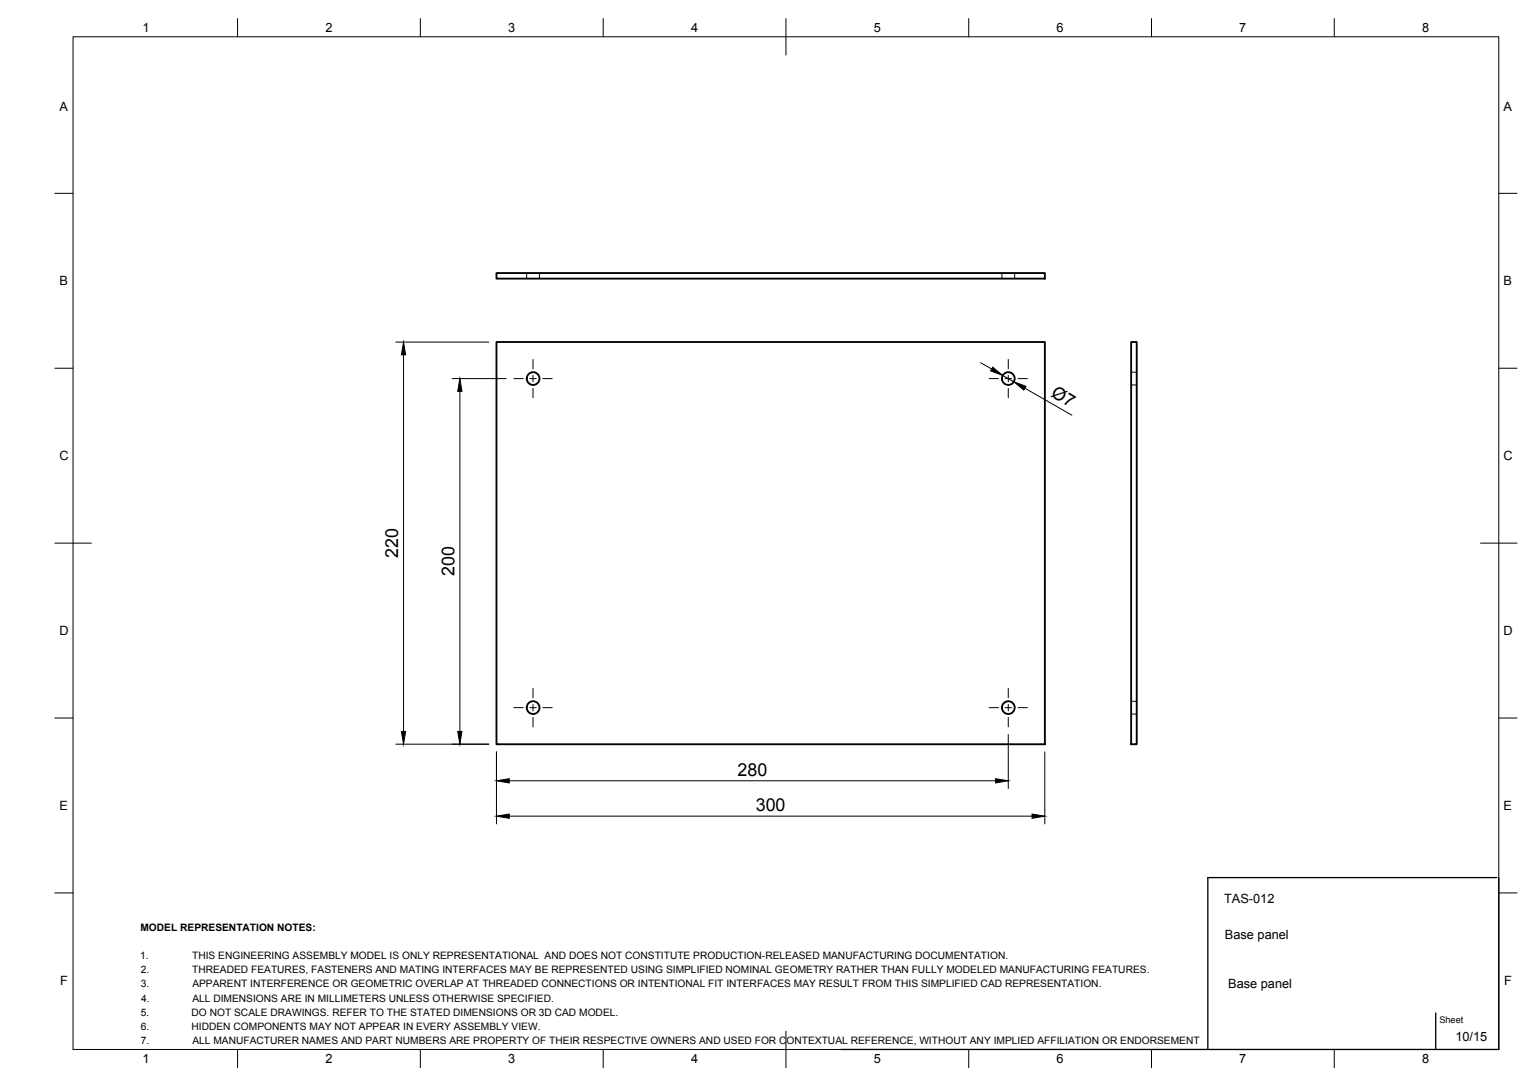
ISO-10303-21;
HEADER;
/* Generated by software containing ST-Developer
 * from STEP Tools, Inc. (www.steptools.com) 
 */

FILE_DESCRIPTION(
/* description */ (
'Independent welded steel electronics enclosure with removable sealed 
lid, internal mounting tray and two threaded cable entries. 300 x 220 
mm body. No ingress or electrical safety rating assigned.'),
/* implementation_level */ '2;1');

FILE_NAME(
/* name */ 'Base panel.step',
/* time_stamp */ '2026-11-14T09:13:27-08:00',
/* author */ (''),
/* organization */ (''),
/* preprocessor_version */ 'ST-DEVELOPER v20.2',
/* originating_system */ 'Autodesk Translation Framework v15.17.0.0',
/* authorisation */ '');

FILE_SCHEMA (('AUTOMOTIVE_DESIGN { 1 0 10303 214 3 1 1 }'));
ENDSEC;

DATA;
#10=MECHANICAL_DESIGN_GEOMETRIC_PRESENTATION_REPRESENTATION('',(#966),#94412);
#936=SHAPE_REPRESENTATION_RELATIONSHIP('SRR','None',#94488,#951);
#951=ADVANCED_BREP_SHAPE_REPRESENTATION('',(#981),#94397);
#966=STYLED_ITEM('',(#94576),#981);
#981=MANIFOLD_SOLID_BREP('Body1',#8251);
#996=FACE_BOUND('',#1523,.T.);
#997=FACE_BOUND('',#1524,.T.);
#998=FACE_BOUND('',#1525,.T.);
#999=FACE_BOUND('',#1526,.T.);
#1000=FACE_BOUND('',#1528,.T.);
#1001=FACE_BOUND('',#1529,.T.);
#1002=FACE_BOUND('',#1530,.T.);
#1003=FACE_BOUND('',#1531,.T.);
#1058=PLANE('',#8447);
#1059=PLANE('',#8448);
#1060=PLANE('',#8449);
#1061=PLANE('',#8450);
#1062=PLANE('',#8451);
#1063=PLANE('',#8452);
#1158=FACE_OUTER_BOUND('',#1514,.T.);
#1159=FACE_OUTER_BOUND('',#1515,.T.);
#1160=FACE_OUTER_BOUND('',#1516,.T.);
#1161=FACE_OUTER_BOUND('',#1517,.T.);
#1162=FACE_OUTER_BOUND('',#1518,.T.);
#1163=FACE_OUTER_BOUND('',#1519,.T.);
#1164=FACE_OUTER_BOUND('',#1520,.T.);
#1165=FACE_OUTER_BOUND('',#1521,.T.);
#1166=FACE_OUTER_BOUND('',#1522,.T.);
#1167=FACE_OUTER_BOUND('',#1527,.T.);
#1514=EDGE_LOOP('',(#5094,#5095,#5096,#5097));
#1515=EDGE_LOOP('',(#5098,#5099,#5100,#5101));
#1516=EDGE_LOOP('',(#5102,#5103,#5104,#5105));
#1517=EDGE_LOOP('',(#5106,#5107,#5108,#5109));
#1518=EDGE_LOOP('',(#5110,#5111,#5112,#5113));
#1519=EDGE_LOOP('',(#5114,#5115,#5116,#5117));
#1520=EDGE_LOOP('',(#5118,#5119,#5120,#5121));
#1521=EDGE_LOOP('',(#5122,#5123,#5124,#5125));
#1522=EDGE_LOOP('',(#5126,#5127,#5128,#5129));
#1523=EDGE_LOOP('',(#5130));
#1524=EDGE_LOOP('',(#5131));
#1525=EDGE_LOOP('',(#5132));
#1526=EDGE_LOOP('',(#5133));
#1527=EDGE_LOOP('',(#5134,#5135,#5136,#5137));
#1528=EDGE_LOOP('',(#5138));
#1529=EDGE_LOOP('',(#5139));
#1530=EDGE_LOOP('',(#5140));
#1531=EDGE_LOOP('',(#5141));
#1932=LINE('',#10367,#2330);
#1933=LINE('',#10373,#2331);
#1934=LINE('',#10379,#2332);
#1935=LINE('',#10385,#2333);
#1936=LINE('',#10390,#2334);
#1937=LINE('',#10392,#2335);
#1938=LINE('',#10394,#2336);
#1939=LINE('',#10395,#2337);
#1940=LINE('',#10398,#2338);
#1941=LINE('',#10400,#2339);
#1942=LINE('',#10401,#2340);
#1943=LINE('',#10404,#2341);
#1944=LINE('',#10406,#2342);
#1945=LINE('',#10407,#2343);
#1946=LINE('',#10409,#2344);
#1947=LINE('',#10410,#2345);
#2330=VECTOR('',#8952,3.5);
#2331=VECTOR('',#8959,3.5);
#2332=VECTOR('',#8966,3.5);
#2333=VECTOR('',#8973,3.5);
#2334=VECTOR('',#8978,10.);
#2335=VECTOR('',#8979,10.);
#2336=VECTOR('',#8980,10.);
#2337=VECTOR('',#8981,10.);
#2338=VECTOR('',#8984,10.);
#2339=VECTOR('',#8985,10.);
#2340=VECTOR('',#8986,10.);
#2341=VECTOR('',#8989,10.);
#2342=VECTOR('',#8990,10.);
#2343=VECTOR('',#8991,10.);
#2344=VECTOR('',#8994,10.);
#2345=VECTOR('',#8995,10.);
#2728=CIRCLE('',#8436,3.5);
#2729=CIRCLE('',#8437,3.5);
#2730=CIRCLE('',#8439,3.5);
#2731=CIRCLE('',#8440,3.5);
#2732=CIRCLE('',#8442,3.5);
#2733=CIRCLE('',#8443,3.5);
#2734=CIRCLE('',#8445,3.5);
#2735=CIRCLE('',#8446,3.5);
#2846=VERTEX_POINT('',#10364);
#2847=VERTEX_POINT('',#10366);
#2848=VERTEX_POINT('',#10370);
#2849=VERTEX_POINT('',#10372);
#2850=VERTEX_POINT('',#10376);
#2851=VERTEX_POINT('',#10378);
#2852=VERTEX_POINT('',#10382);
#2853=VERTEX_POINT('',#10384);
#2854=VERTEX_POINT('',#10388);
#2855=VERTEX_POINT('',#10389);
#2856=VERTEX_POINT('',#10391);
#2857=VERTEX_POINT('',#10393);
#2858=VERTEX_POINT('',#10397);
#2859=VERTEX_POINT('',#10399);
#2860=VERTEX_POINT('',#10403);
#2861=VERTEX_POINT('',#10405);
#3812=EDGE_CURVE('',#2846,#2846,#2728,.T.);
#3813=EDGE_CURVE('',#2846,#2847,#1932,.T.);
#3814=EDGE_CURVE('',#2847,#2847,#2729,.T.);
#3815=EDGE_CURVE('',#2848,#2848,#2730,.T.);
#3816=EDGE_CURVE('',#2848,#2849,#1933,.T.);
#3817=EDGE_CURVE('',#2849,#2849,#2731,.T.);
#3818=EDGE_CURVE('',#2850,#2850,#2732,.T.);
#3819=EDGE_CURVE('',#2850,#2851,#1934,.T.);
#3820=EDGE_CURVE('',#2851,#2851,#2733,.T.);
#3821=EDGE_CURVE('',#2852,#2852,#2734,.T.);
#3822=EDGE_CURVE('',#2852,#2853,#1935,.T.);
#3823=EDGE_CURVE('',#2853,#2853,#2735,.T.);
#3824=EDGE_CURVE('',#2854,#2855,#1936,.T.);
#3825=EDGE_CURVE('',#2855,#2856,#1937,.T.);
#3826=EDGE_CURVE('',#2857,#2856,#1938,.T.);
#3827=EDGE_CURVE('',#2854,#2857,#1939,.T.);
#3828=EDGE_CURVE('',#2858,#2854,#1940,.T.);
#3829=EDGE_CURVE('',#2859,#2857,#1941,.T.);
#3830=EDGE_CURVE('',#2858,#2859,#1942,.T.);
#3831=EDGE_CURVE('',#2860,#2858,#1943,.T.);
#3832=EDGE_CURVE('',#2861,#2859,#1944,.T.);
#3833=EDGE_CURVE('',#2860,#2861,#1945,.T.);
#3834=EDGE_CURVE('',#2855,#2860,#1946,.T.);
#3835=EDGE_CURVE('',#2856,#2861,#1947,.T.);
#5094=ORIENTED_EDGE('',*,*,#3812,.F.);
#5095=ORIENTED_EDGE('',*,*,#3813,.T.);
#5096=ORIENTED_EDGE('',*,*,#3814,.F.);
#5097=ORIENTED_EDGE('',*,*,#3813,.F.);
#5098=ORIENTED_EDGE('',*,*,#3815,.F.);
#5099=ORIENTED_EDGE('',*,*,#3816,.T.);
#5100=ORIENTED_EDGE('',*,*,#3817,.F.);
#5101=ORIENTED_EDGE('',*,*,#3816,.F.);
#5102=ORIENTED_EDGE('',*,*,#3818,.F.);
#5103=ORIENTED_EDGE('',*,*,#3819,.T.);
#5104=ORIENTED_EDGE('',*,*,#3820,.F.);
#5105=ORIENTED_EDGE('',*,*,#3819,.F.);
#5106=ORIENTED_EDGE('',*,*,#3821,.F.);
#5107=ORIENTED_EDGE('',*,*,#3822,.T.);
#5108=ORIENTED_EDGE('',*,*,#3823,.F.);
#5109=ORIENTED_EDGE('',*,*,#3822,.F.);
#5110=ORIENTED_EDGE('',*,*,#3824,.T.);
#5111=ORIENTED_EDGE('',*,*,#3825,.T.);
#5112=ORIENTED_EDGE('',*,*,#3826,.F.);
#5113=ORIENTED_EDGE('',*,*,#3827,.F.);
#5114=ORIENTED_EDGE('',*,*,#3828,.T.);
#5115=ORIENTED_EDGE('',*,*,#3827,.T.);
#5116=ORIENTED_EDGE('',*,*,#3829,.F.);
#5117=ORIENTED_EDGE('',*,*,#3830,.F.);
#5118=ORIENTED_EDGE('',*,*,#3831,.T.);
#5119=ORIENTED_EDGE('',*,*,#3830,.T.);
#5120=ORIENTED_EDGE('',*,*,#3832,.F.);
#5121=ORIENTED_EDGE('',*,*,#3833,.F.);
#5122=ORIENTED_EDGE('',*,*,#3834,.T.);
#5123=ORIENTED_EDGE('',*,*,#3833,.T.);
#5124=ORIENTED_EDGE('',*,*,#3835,.F.);
#5125=ORIENTED_EDGE('',*,*,#3825,.F.);
#5126=ORIENTED_EDGE('',*,*,#3835,.T.);
#5127=ORIENTED_EDGE('',*,*,#3832,.T.);
#5128=ORIENTED_EDGE('',*,*,#3829,.T.);
#5129=ORIENTED_EDGE('',*,*,#3826,.T.);
#5130=ORIENTED_EDGE('',*,*,#3812,.T.);
#5131=ORIENTED_EDGE('',*,*,#3815,.T.);
#5132=ORIENTED_EDGE('',*,*,#3818,.T.);
#5133=ORIENTED_EDGE('',*,*,#3821,.T.);
#5134=ORIENTED_EDGE('',*,*,#3834,.F.);
#5135=ORIENTED_EDGE('',*,*,#3824,.F.);
#5136=ORIENTED_EDGE('',*,*,#3828,.F.);
#5137=ORIENTED_EDGE('',*,*,#3831,.F.);
#5138=ORIENTED_EDGE('',*,*,#3814,.T.);
#5139=ORIENTED_EDGE('',*,*,#3817,.T.);
#5140=ORIENTED_EDGE('',*,*,#3820,.T.);
#5141=ORIENTED_EDGE('',*,*,#3823,.T.);
#7658=CYLINDRICAL_SURFACE('',#8435,3.5);
#7659=CYLINDRICAL_SURFACE('',#8438,3.5);
#7660=CYLINDRICAL_SURFACE('',#8441,3.5);
#7661=CYLINDRICAL_SURFACE('',#8444,3.5);
#7895=ADVANCED_FACE('',(#1158),#7658,.F.);
#7896=ADVANCED_FACE('',(#1159),#7659,.F.);
#7897=ADVANCED_FACE('',(#1160),#7660,.F.);
#7898=ADVANCED_FACE('',(#1161),#7661,.F.);
#7899=ADVANCED_FACE('',(#1162),#1058,.T.);
#7900=ADVANCED_FACE('',(#1163),#1059,.T.);
#7901=ADVANCED_FACE('',(#1164),#1060,.T.);
#7902=ADVANCED_FACE('',(#1165),#1061,.T.);
#7903=ADVANCED_FACE('',(#1166,#996,#997,#998,#999),#1062,.T.);
#7904=ADVANCED_FACE('',(#1167,#1000,#1001,#1002,#1003),#1063,.F.);
#8251=CLOSED_SHELL('',(#7895,#7896,#7897,#7898,#7899,#7900,#7901,#7902,
#7903,#7904));
#8434=AXIS2_PLACEMENT_3D('',#10362,#8946,#8947);
#8435=AXIS2_PLACEMENT_3D('',#10363,#8948,#8949);
#8436=AXIS2_PLACEMENT_3D('',#10365,#8950,#8951);
#8437=AXIS2_PLACEMENT_3D('',#10368,#8953,#8954);
#8438=AXIS2_PLACEMENT_3D('',#10369,#8955,#8956);
#8439=AXIS2_PLACEMENT_3D('',#10371,#8957,#8958);
#8440=AXIS2_PLACEMENT_3D('',#10374,#8960,#8961);
#8441=AXIS2_PLACEMENT_3D('',#10375,#8962,#8963);
#8442=AXIS2_PLACEMENT_3D('',#10377,#8964,#8965);
#8443=AXIS2_PLACEMENT_3D('',#10380,#8967,#8968);
#8444=AXIS2_PLACEMENT_3D('',#10381,#8969,#8970);
#8445=AXIS2_PLACEMENT_3D('',#10383,#8971,#8972);
#8446=AXIS2_PLACEMENT_3D('',#10386,#8974,#8975);
#8447=AXIS2_PLACEMENT_3D('',#10387,#8976,#8977);
#8448=AXIS2_PLACEMENT_3D('',#10396,#8982,#8983);
#8449=AXIS2_PLACEMENT_3D('',#10402,#8987,#8988);
#8450=AXIS2_PLACEMENT_3D('',#10408,#8992,#8993);
#8451=AXIS2_PLACEMENT_3D('',#10411,#8996,#8997);
#8452=AXIS2_PLACEMENT_3D('',#10412,#8998,#8999);
#8946=DIRECTION('axis',(0.,0.,1.));
#8947=DIRECTION('refdir',(1.,0.,0.));
#8948=DIRECTION('center_axis',(0.,0.,-1.));
#8949=DIRECTION('ref_axis',(1.,0.,0.));
#8950=DIRECTION('center_axis',(0.,0.,-1.));
#8951=DIRECTION('ref_axis',(1.,0.,0.));
#8952=DIRECTION('',(0.,0.,-1.));
#8953=DIRECTION('center_axis',(0.,0.,1.));
#8954=DIRECTION('ref_axis',(1.,0.,0.));
#8955=DIRECTION('center_axis',(0.,0.,-1.));
#8956=DIRECTION('ref_axis',(1.,0.,0.));
#8957=DIRECTION('center_axis',(0.,0.,-1.));
#8958=DIRECTION('ref_axis',(1.,0.,0.));
#8959=DIRECTION('',(0.,0.,-1.));
#8960=DIRECTION('center_axis',(0.,0.,1.));
#8961=DIRECTION('ref_axis',(1.,0.,0.));
#8962=DIRECTION('center_axis',(0.,0.,-1.));
#8963=DIRECTION('ref_axis',(1.,0.,0.));
#8964=DIRECTION('center_axis',(0.,0.,-1.));
#8965=DIRECTION('ref_axis',(1.,0.,0.));
#8966=DIRECTION('',(0.,0.,-1.));
#8967=DIRECTION('center_axis',(0.,0.,1.));
#8968=DIRECTION('ref_axis',(1.,0.,0.));
#8969=DIRECTION('center_axis',(0.,0.,-1.));
#8970=DIRECTION('ref_axis',(1.,0.,0.));
#8971=DIRECTION('center_axis',(0.,0.,-1.));
#8972=DIRECTION('ref_axis',(1.,0.,0.));
#8973=DIRECTION('',(0.,0.,-1.));
#8974=DIRECTION('center_axis',(0.,0.,1.));
#8975=DIRECTION('ref_axis',(1.,0.,0.));
#8976=DIRECTION('center_axis',(0.,1.,0.));
#8977=DIRECTION('ref_axis',(-1.,0.,0.));
#8978=DIRECTION('',(-1.,0.,0.));
#8979=DIRECTION('',(0.,0.,1.));
#8980=DIRECTION('',(-1.,0.,0.));
#8981=DIRECTION('',(0.,0.,1.));
#8982=DIRECTION('center_axis',(1.,0.,0.));
#8983=DIRECTION('ref_axis',(0.,1.,0.));
#8984=DIRECTION('',(0.,1.,0.));
#8985=DIRECTION('',(0.,1.,0.));
#8986=DIRECTION('',(0.,0.,1.));
#8987=DIRECTION('center_axis',(0.,-1.,0.));
#8988=DIRECTION('ref_axis',(1.,0.,0.));
#8989=DIRECTION('',(1.,0.,0.));
#8990=DIRECTION('',(1.,0.,0.));
#8991=DIRECTION('',(0.,0.,1.));
#8992=DIRECTION('center_axis',(-1.,0.,0.));
#8993=DIRECTION('ref_axis',(0.,-1.,0.));
#8994=DIRECTION('',(0.,-1.,0.));
#8995=DIRECTION('',(0.,-1.,0.));
#8996=DIRECTION('center_axis',(0.,0.,1.));
#8997=DIRECTION('ref_axis',(1.,0.,0.));
#8998=DIRECTION('center_axis',(0.,0.,1.));
#8999=DIRECTION('ref_axis',(1.,0.,0.));
#10362=CARTESIAN_POINT('',(0.,0.,0.));
#10363=CARTESIAN_POINT('Origin',(130.,-90.,1.5));
#10364=CARTESIAN_POINT('',(126.5,-90.,3.));
#10365=CARTESIAN_POINT('Origin',(130.,-90.,3.));
#10366=CARTESIAN_POINT('',(126.5,-90.,0.));
#10367=CARTESIAN_POINT('',(126.5,-90.,1.5));
#10368=CARTESIAN_POINT('Origin',(130.,-90.,0.));
#10369=CARTESIAN_POINT('Origin',(-130.,-90.,1.5));
#10370=CARTESIAN_POINT('',(-133.5,-90.,3.));
#10371=CARTESIAN_POINT('Origin',(-130.,-90.,3.));
#10372=CARTESIAN_POINT('',(-133.5,-90.,0.));
#10373=CARTESIAN_POINT('',(-133.5,-90.,1.5));
#10374=CARTESIAN_POINT('Origin',(-130.,-90.,0.));
#10375=CARTESIAN_POINT('Origin',(-130.,90.,1.5));
#10376=CARTESIAN_POINT('',(-133.5,90.,3.));
#10377=CARTESIAN_POINT('Origin',(-130.,90.,3.));
#10378=CARTESIAN_POINT('',(-133.5,90.,0.));
#10379=CARTESIAN_POINT('',(-133.5,90.,1.5));
#10380=CARTESIAN_POINT('Origin',(-130.,90.,0.));
#10381=CARTESIAN_POINT('Origin',(130.,90.,1.5));
#10382=CARTESIAN_POINT('',(126.5,90.,3.));
#10383=CARTESIAN_POINT('Origin',(130.,90.,3.));
#10384=CARTESIAN_POINT('',(126.5,90.,0.));
#10385=CARTESIAN_POINT('',(126.5,90.,1.5));
#10386=CARTESIAN_POINT('Origin',(130.,90.,0.));
#10387=CARTESIAN_POINT('Origin',(150.,110.,0.));
#10388=CARTESIAN_POINT('',(150.,110.,0.));
#10389=CARTESIAN_POINT('',(-150.,110.,0.));
#10390=CARTESIAN_POINT('',(150.,110.,0.));
#10391=CARTESIAN_POINT('',(-150.,110.,3.));
#10392=CARTESIAN_POINT('',(-150.,110.,0.));
#10393=CARTESIAN_POINT('',(150.,110.,3.));
#10394=CARTESIAN_POINT('',(150.,110.,3.));
#10395=CARTESIAN_POINT('',(150.,110.,0.));
#10396=CARTESIAN_POINT('Origin',(150.,-110.,0.));
#10397=CARTESIAN_POINT('',(150.,-110.,0.));
#10398=CARTESIAN_POINT('',(150.,-110.,0.));
#10399=CARTESIAN_POINT('',(150.,-110.,3.));
#10400=CARTESIAN_POINT('',(150.,-110.,3.));
#10401=CARTESIAN_POINT('',(150.,-110.,0.));
#10402=CARTESIAN_POINT('Origin',(-150.,-110.,0.));
#10403=CARTESIAN_POINT('',(-150.,-110.,0.));
#10404=CARTESIAN_POINT('',(-150.,-110.,0.));
#10405=CARTESIAN_POINT('',(-150.,-110.,3.));
#10406=CARTESIAN_POINT('',(-150.,-110.,3.));
#10407=CARTESIAN_POINT('',(-150.,-110.,0.));
#10408=CARTESIAN_POINT('Origin',(-150.,110.,0.));
#10409=CARTESIAN_POINT('',(-150.,110.,0.));
#10410=CARTESIAN_POINT('',(-150.,110.,3.));
#10411=CARTESIAN_POINT('Origin',(0.,0.,3.));
#10412=CARTESIAN_POINT('Origin',(0.,0.,0.));
#94379=UNCERTAINTY_MEASURE_WITH_UNIT(LENGTH_MEASURE(0.01),#94413,
'DISTANCE_ACCURACY_VALUE',
'Maximum model space distance between geometric entities at asserted c
onnectivities');
#94394=UNCERTAINTY_MEASURE_WITH_UNIT(LENGTH_MEASURE(0.01),#94413,
'DISTANCE_ACCURACY_VALUE',
'Maximum model space distance between geometric entities at asserted c
onnectivities');
#94397=(
GEOMETRIC_REPRESENTATION_CONTEXT(3)
GLOBAL_UNCERTAINTY_ASSIGNED_CONTEXT((#94379))
GLOBAL_UNIT_ASSIGNED_CONTEXT((#94413,#94415,#94416))
REPRESENTATION_CONTEXT('','3D')
);
#94412=(
GEOMETRIC_REPRESENTATION_CONTEXT(3)
GLOBAL_UNCERTAINTY_ASSIGNED_CONTEXT((#94394))
GLOBAL_UNIT_ASSIGNED_CONTEXT((#94413,#94415,#94416))
REPRESENTATION_CONTEXT('','3D')
);
#94413=(
LENGTH_UNIT()
NAMED_UNIT(*)
SI_UNIT(.MILLI.,.METRE.)
);
#94415=(
NAMED_UNIT(*)
PLANE_ANGLE_UNIT()
SI_UNIT($,.RADIAN.)
);
#94416=(
NAMED_UNIT(*)
SI_UNIT($,.STERADIAN.)
SOLID_ANGLE_UNIT()
);
#94419=SHAPE_DEFINITION_REPRESENTATION(#94436,#94488);
#94436=PRODUCT_DEFINITION_SHAPE('',$,#94506);
#94488=SHAPE_REPRESENTATION('',(#8434),#94397);
#94503=PRODUCT_DEFINITION_CONTEXT('part definition',#94556,'design');
#94506=PRODUCT_DEFINITION('Base panel','Base panel',#94523,#94503);
#94523=PRODUCT_DEFINITION_FORMATION('',$,#94560);
#94556=APPLICATION_CONTEXT(
'Core Data for Automotive Mechanical Design Process');
#94557=PRODUCT_CONTEXT('part definition',#94556,'mechanical');
#94560=PRODUCT('Base panel','Base panel',
'3 mm steel sheet; weld adjoining shell-panel edges continuously. Fabr
ication weld specification remains to be selected.',(#94557));
#94576=PRESENTATION_STYLE_ASSIGNMENT((#94583));
#94583=SURFACE_STYLE_USAGE(.BOTH.,#94590);
#94590=SURFACE_SIDE_STYLE('',(#94597));
#94597=SURFACE_STYLE_FILL_AREA(#94604);
#94604=FILL_AREA_STYLE('Opaque(23,69,131)',(#94611));
#94611=FILL_AREA_STYLE_COLOUR('Opaque(23,69,131)',#94618);
#94618=COLOUR_RGB('Opaque(23,69,131)',0.0901960784313725,0.270588235294118,
0.513725490196078);
ENDSEC;
END-ISO-10303-21;
